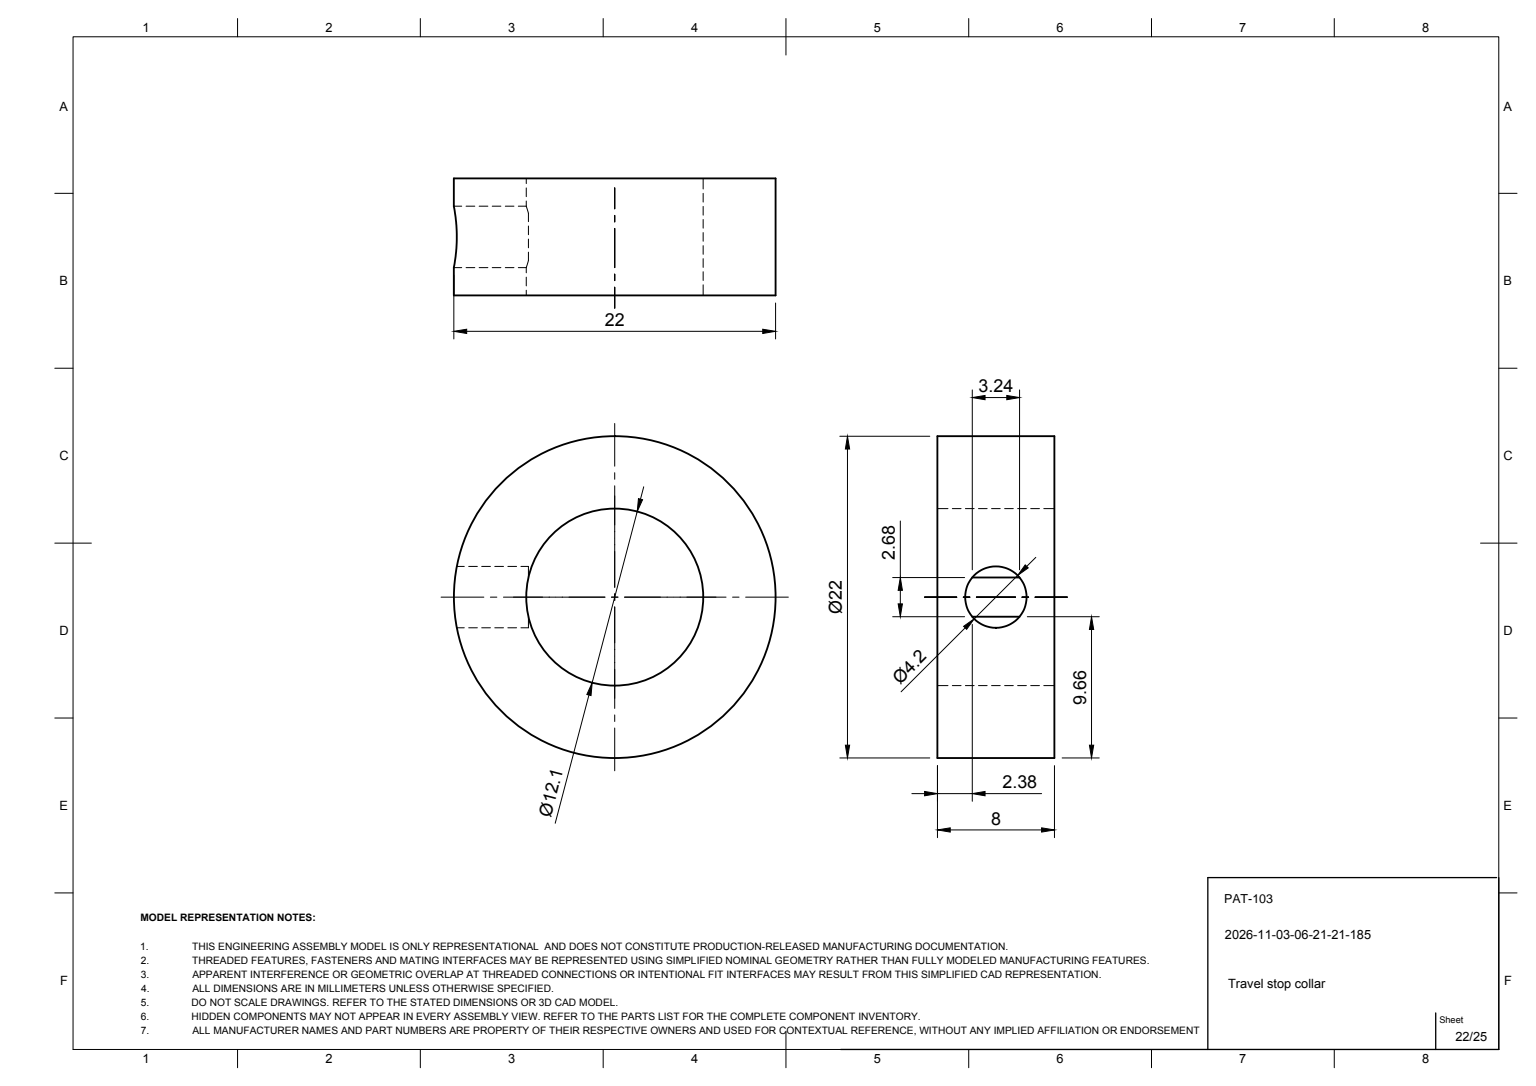
ISO-10303-21;
HEADER;
/* Generated by software containing ST-Developer
 * from STEP Tools, Inc. (www.steptools.com) 
 */

FILE_DESCRIPTION(
/* description */ ('Telescoping shaft support with lock collar'),
/* implementation_level */ '2;1');

FILE_NAME(
/* name */ 'Travel stop collar.step',
/* time_stamp */ '2026-10-27T10:48:51-07:00',
/* author */ (''),
/* organization */ (''),
/* preprocessor_version */ 'ST-DEVELOPER v20.2',
/* originating_system */ 'Autodesk Translation Framework v15.17.0.0',
/* authorisation */ '');

FILE_SCHEMA (('AUTOMOTIVE_DESIGN { 1 0 10303 214 3 1 1 }'));
ENDSEC;

DATA;
#10=MECHANICAL_DESIGN_GEOMETRIC_PRESENTATION_REPRESENTATION('',(#255),#7349);
#187=B_SPLINE_CURVE_WITH_KNOTS('',3,(#6910,#6911,#6912,#6913,#6914,#6915),
 .UNSPECIFIED.,.F.,.F.,(4,2,4),(0.818088904349175,0.878131747417171,0.957937926194042),
 .UNSPECIFIED.);
#188=B_SPLINE_CURVE_WITH_KNOTS('',3,(#6919,#6920,#6921,#6922,#6923,#6924),
 .UNSPECIFIED.,.F.,.F.,(4,2,4),(0.319312642064681,0.399118820841551,0.459161663909547),
 .UNSPECIFIED.);
#189=B_SPLINE_CURVE_WITH_KNOTS('',3,(#6925,#6926,#6927,#6928,#6929,#6930),
 .UNSPECIFIED.,.F.,.F.,(4,2,4),(0.179463620219814,0.23950646328781,0.319312642064681),
 .UNSPECIFIED.);
#190=B_SPLINE_CURVE_WITH_KNOTS('',3,(#6931,#6932,#6933,#6934,#6935,#6936),
 .UNSPECIFIED.,.F.,.F.,(4,2,4),(0.957937926194042,1.03774410497091,1.09778694803891),
 .UNSPECIFIED.);
#191=B_SPLINE_CURVE_WITH_KNOTS('',3,(#6940,#6941,#6942,#6943,#6944,#6945,
#6946,#6947,#6948,#6949),.UNSPECIFIED.,.F.,.F.,(4,2,2,2,4),(0.,0.0793157643915228,
0.158631528783046,0.237943615933651,0.317255703084257),.UNSPECIFIED.);
#192=B_SPLINE_CURVE_WITH_KNOTS('',3,(#6951,#6952,#6953,#6954,#6955,#6956,
#6957,#6958,#6959,#6960),.UNSPECIFIED.,.F.,.F.,(4,2,2,2,4),(0.951767109252772,
1.03107919640338,1.11039128355398,1.18970704794551,1.26902281233703),
 .UNSPECIFIED.);
#193=B_SPLINE_CURVE_WITH_KNOTS('',3,(#6961,#6962,#6963,#6964,#6965,#6966,
#6967,#6968,#6969,#6970,#6971,#6972,#6973,#6974,#6975,#6976,#6977,#6978),
 .UNSPECIFIED.,.F.,.F.,(4,2,2,2,2,2,2,2,4),(0.317255703084257,0.396567790234863,
0.475879877385469,0.555195641776992,0.634511406168514,0.713827170560037,
0.79314293495156,0.872455022102166,0.951767109252772),.UNSPECIFIED.);
#215=SHAPE_REPRESENTATION_RELATIONSHIP('SRR','None',#7459,#235);
#235=ADVANCED_BREP_SHAPE_REPRESENTATION('',(#274),#7343);
#255=STYLED_ITEM('',(#7641),#274);
#274=MANIFOLD_SOLID_BREP('Body1',#3979);
#349=FACE_BOUND('',#967,.T.);
#350=FACE_BOUND('',#969,.T.);
#461=PLANE('',#4573);
#462=PLANE('',#4577);
#463=PLANE('',#4584);
#464=PLANE('',#4585);
#665=FACE_OUTER_BOUND('',#961,.T.);
#666=FACE_OUTER_BOUND('',#962,.T.);
#667=FACE_OUTER_BOUND('',#963,.T.);
#668=FACE_OUTER_BOUND('',#964,.T.);
#669=FACE_OUTER_BOUND('',#965,.T.);
#670=FACE_OUTER_BOUND('',#966,.T.);
#671=FACE_OUTER_BOUND('',#968,.T.);
#961=EDGE_LOOP('',(#3428,#3429));
#962=EDGE_LOOP('',(#3430,#3431,#3432,#3433,#3434,#3435,#3436,#3437,#3438,
#3439,#3440));
#963=EDGE_LOOP('',(#3441,#3442));
#964=EDGE_LOOP('',(#3443,#3444,#3445,#3446,#3447,#3448,#3449,#3450,#3451,
#3452,#3453,#3454));
#965=EDGE_LOOP('',(#3455,#3456,#3457,#3458,#3459,#3460,#3461,#3462,#3463));
#966=EDGE_LOOP('',(#3464));
#967=EDGE_LOOP('',(#3465));
#968=EDGE_LOOP('',(#3466));
#969=EDGE_LOOP('',(#3467));
#1241=LINE('',#6905,#1521);
#1242=LINE('',#6938,#1522);
#1243=LINE('',#6980,#1523);
#1244=LINE('',#6984,#1524);
#1245=LINE('',#6986,#1525);
#1246=LINE('',#6991,#1526);
#1247=LINE('',#6993,#1527);
#1521=VECTOR('',#5655,1.);
#1522=VECTOR('',#5662,0.210000000000001);
#1523=VECTOR('',#5665,1.);
#1524=VECTOR('',#5670,0.605);
#1525=VECTOR('',#5671,0.605);
#1526=VECTOR('',#5678,1.1);
#1527=VECTOR('',#5679,1.1);
#1762=CIRCLE('',#4574,0.210000000000001);
#1763=CIRCLE('',#4576,0.210000000000001);
#1764=CIRCLE('',#4579,0.605);
#1765=CIRCLE('',#4580,0.605);
#1766=CIRCLE('',#4582,1.1);
#1767=CIRCLE('',#4583,1.1);
#2059=VERTEX_POINT('',#6903);
#2060=VERTEX_POINT('',#6904);
#2061=VERTEX_POINT('',#6908);
#2062=VERTEX_POINT('',#6909);
#2063=VERTEX_POINT('',#6916);
#2064=VERTEX_POINT('',#6918);
#2065=VERTEX_POINT('',#6937);
#2066=VERTEX_POINT('',#6939);
#2067=VERTEX_POINT('',#6950);
#2068=VERTEX_POINT('',#6982);
#2069=VERTEX_POINT('',#6985);
#2070=VERTEX_POINT('',#6989);
#2071=VERTEX_POINT('',#6992);
#2526=EDGE_CURVE('',#2059,#2060,#1241,.T.);
#2527=EDGE_CURVE('',#2059,#2060,#1762,.T.);
#2528=EDGE_CURVE('',#2061,#2062,#187,.T.);
#2529=EDGE_CURVE('',#2063,#2061,#1763,.T.);
#2530=EDGE_CURVE('',#2064,#2063,#188,.T.);
#2531=EDGE_CURVE('',#2060,#2064,#189,.T.);
#2532=EDGE_CURVE('',#2062,#2059,#190,.T.);
#2533=EDGE_CURVE('',#2062,#2065,#1242,.T.);
#2534=EDGE_CURVE('',#2066,#2065,#191,.T.);
#2535=EDGE_CURVE('',#2067,#2066,#192,.T.);
#2536=EDGE_CURVE('',#2065,#2067,#193,.T.);
#2537=EDGE_CURVE('',#2063,#2061,#1243,.T.);
#2538=EDGE_CURVE('',#2068,#2068,#1764,.T.);
#2539=EDGE_CURVE('',#2068,#2064,#1244,.T.);
#2540=EDGE_CURVE('',#2062,#2069,#1245,.T.);
#2541=EDGE_CURVE('',#2069,#2069,#1765,.T.);
#2542=EDGE_CURVE('',#2070,#2070,#1766,.T.);
#2543=EDGE_CURVE('',#2070,#2067,#1246,.T.);
#2544=EDGE_CURVE('',#2065,#2071,#1247,.T.);
#2545=EDGE_CURVE('',#2071,#2071,#1767,.T.);
#3428=ORIENTED_EDGE('',*,*,#2526,.F.);
#3429=ORIENTED_EDGE('',*,*,#2527,.T.);
#3430=ORIENTED_EDGE('',*,*,#2528,.F.);
#3431=ORIENTED_EDGE('',*,*,#2529,.F.);
#3432=ORIENTED_EDGE('',*,*,#2530,.F.);
#3433=ORIENTED_EDGE('',*,*,#2531,.F.);
#3434=ORIENTED_EDGE('',*,*,#2527,.F.);
#3435=ORIENTED_EDGE('',*,*,#2532,.F.);
#3436=ORIENTED_EDGE('',*,*,#2533,.T.);
#3437=ORIENTED_EDGE('',*,*,#2534,.F.);
#3438=ORIENTED_EDGE('',*,*,#2535,.F.);
#3439=ORIENTED_EDGE('',*,*,#2536,.F.);
#3440=ORIENTED_EDGE('',*,*,#2533,.F.);
#3441=ORIENTED_EDGE('',*,*,#2537,.F.);
#3442=ORIENTED_EDGE('',*,*,#2529,.T.);
#3443=ORIENTED_EDGE('',*,*,#2538,.F.);
#3444=ORIENTED_EDGE('',*,*,#2539,.T.);
#3445=ORIENTED_EDGE('',*,*,#2530,.T.);
#3446=ORIENTED_EDGE('',*,*,#2537,.T.);
#3447=ORIENTED_EDGE('',*,*,#2528,.T.);
#3448=ORIENTED_EDGE('',*,*,#2540,.T.);
#3449=ORIENTED_EDGE('',*,*,#2541,.T.);
#3450=ORIENTED_EDGE('',*,*,#2540,.F.);
#3451=ORIENTED_EDGE('',*,*,#2532,.T.);
#3452=ORIENTED_EDGE('',*,*,#2526,.T.);
#3453=ORIENTED_EDGE('',*,*,#2531,.T.);
#3454=ORIENTED_EDGE('',*,*,#2539,.F.);
#3455=ORIENTED_EDGE('',*,*,#2542,.F.);
#3456=ORIENTED_EDGE('',*,*,#2543,.T.);
#3457=ORIENTED_EDGE('',*,*,#2535,.T.);
#3458=ORIENTED_EDGE('',*,*,#2534,.T.);
#3459=ORIENTED_EDGE('',*,*,#2544,.T.);
#3460=ORIENTED_EDGE('',*,*,#2545,.T.);
#3461=ORIENTED_EDGE('',*,*,#2544,.F.);
#3462=ORIENTED_EDGE('',*,*,#2536,.T.);
#3463=ORIENTED_EDGE('',*,*,#2543,.F.);
#3464=ORIENTED_EDGE('',*,*,#2542,.T.);
#3465=ORIENTED_EDGE('',*,*,#2538,.T.);
#3466=ORIENTED_EDGE('',*,*,#2545,.F.);
#3467=ORIENTED_EDGE('',*,*,#2541,.F.);
#3724=CYLINDRICAL_SURFACE('',#4575,0.210000000000001);
#3725=CYLINDRICAL_SURFACE('',#4578,0.605);
#3726=CYLINDRICAL_SURFACE('',#4581,1.1);
#3908=ADVANCED_FACE('',(#665),#461,.T.);
#3909=ADVANCED_FACE('',(#666),#3724,.F.);
#3910=ADVANCED_FACE('',(#667),#462,.T.);
#3911=ADVANCED_FACE('',(#668),#3725,.F.);
#3912=ADVANCED_FACE('',(#669),#3726,.T.);
#3913=ADVANCED_FACE('',(#670,#349),#463,.T.);
#3914=ADVANCED_FACE('',(#671,#350),#464,.F.);
#3979=CLOSED_SHELL('',(#3908,#3909,#3910,#3911,#3912,#3913,#3914));
#4572=AXIS2_PLACEMENT_3D('',#6901,#5651,#5652);
#4573=AXIS2_PLACEMENT_3D('',#6902,#5653,#5654);
#4574=AXIS2_PLACEMENT_3D('',#6906,#5656,#5657);
#4575=AXIS2_PLACEMENT_3D('',#6907,#5658,#5659);
#4576=AXIS2_PLACEMENT_3D('',#6917,#5660,#5661);
#4577=AXIS2_PLACEMENT_3D('',#6979,#5663,#5664);
#4578=AXIS2_PLACEMENT_3D('',#6981,#5666,#5667);
#4579=AXIS2_PLACEMENT_3D('',#6983,#5668,#5669);
#4580=AXIS2_PLACEMENT_3D('',#6987,#5672,#5673);
#4581=AXIS2_PLACEMENT_3D('',#6988,#5674,#5675);
#4582=AXIS2_PLACEMENT_3D('',#6990,#5676,#5677);
#4583=AXIS2_PLACEMENT_3D('',#6994,#5680,#5681);
#4584=AXIS2_PLACEMENT_3D('',#6995,#5682,#5683);
#4585=AXIS2_PLACEMENT_3D('',#6996,#5684,#5685);
#5651=DIRECTION('axis',(0.,0.,1.));
#5652=DIRECTION('refdir',(1.,0.,0.));
#5653=DIRECTION('center_axis',(0.,0.,1.));
#5654=DIRECTION('ref_axis',(1.,0.,0.));
#5655=DIRECTION('',(1.,0.,0.));
#5656=DIRECTION('center_axis',(0.,0.,1.));
#5657=DIRECTION('ref_axis',(1.,0.,0.));
#5658=DIRECTION('center_axis',(0.,0.,1.));
#5659=DIRECTION('ref_axis',(1.,0.,0.));
#5660=DIRECTION('center_axis',(0.,0.,1.));
#5661=DIRECTION('ref_axis',(1.,0.,0.));
#5662=DIRECTION('',(0.,0.,1.));
#5663=DIRECTION('center_axis',(0.,0.,1.));
#5664=DIRECTION('ref_axis',(1.,0.,0.));
#5665=DIRECTION('',(-1.,0.,0.));
#5666=DIRECTION('center_axis',(1.,0.,0.));
#5667=DIRECTION('ref_axis',(0.,0.,-1.));
#5668=DIRECTION('center_axis',(-1.,0.,0.));
#5669=DIRECTION('ref_axis',(0.,0.,-1.));
#5670=DIRECTION('',(-1.,0.,0.));
#5671=DIRECTION('',(-1.,0.,0.));
#5672=DIRECTION('center_axis',(-1.,0.,0.));
#5673=DIRECTION('ref_axis',(0.,0.,-1.));
#5674=DIRECTION('center_axis',(1.,0.,0.));
#5675=DIRECTION('ref_axis',(0.,0.,-1.));
#5676=DIRECTION('center_axis',(1.,0.,0.));
#5677=DIRECTION('ref_axis',(0.,0.,-1.));
#5678=DIRECTION('',(-1.,0.,0.));
#5679=DIRECTION('',(-1.,0.,0.));
#5680=DIRECTION('center_axis',(1.,0.,0.));
#5681=DIRECTION('ref_axis',(0.,0.,-1.));
#5682=DIRECTION('center_axis',(1.,0.,0.));
#5683=DIRECTION('ref_axis',(0.,0.,-1.));
#5684=DIRECTION('center_axis',(1.,0.,0.));
#5685=DIRECTION('ref_axis',(0.,0.,-1.));
#6901=CARTESIAN_POINT('',(0.,0.,0.));
#6902=CARTESIAN_POINT('Origin',(-17.3,0.,4.09));
#6903=CARTESIAN_POINT('',(-17.4617868968736,-0.133884278389959,4.09));
#6904=CARTESIAN_POINT('',(-17.1382131031264,-0.133884278389959,4.09));
#6905=CARTESIAN_POINT('',(-17.7,-0.133884278389959,4.09));
#6906=CARTESIAN_POINT('Origin',(-17.3,0.,4.09));
#6907=CARTESIAN_POINT('Origin',(-17.3,0.,4.09));
#6908=CARTESIAN_POINT('',(-17.4617868968736,0.133884278389959,4.09));
#6909=CARTESIAN_POINT('',(-17.51,7.73468293597467E-17,4.105));
#6910=CARTESIAN_POINT('Ctrl Pts',(-17.4617868968736,0.133884278389958,4.09));
#6911=CARTESIAN_POINT('Ctrl Pts',(-17.4747211682176,0.118254395260802,4.09354677224418));
#6912=CARTESIAN_POINT('Ctrl Pts',(-17.4857993165874,0.100109787682302,4.09698224789957));
#6913=CARTESIAN_POINT('Ctrl Pts',(-17.5046385610544,0.0548298721325208,
4.1030741628997));
#6914=CARTESIAN_POINT('Ctrl Pts',(-17.51,0.0266020595922901,4.105));
#6915=CARTESIAN_POINT('Ctrl Pts',(-17.51,-1.73472347597681E-16,4.105));
#6916=CARTESIAN_POINT('',(-17.1382131031264,0.133884278389959,4.09));
#6917=CARTESIAN_POINT('Origin',(-17.3,0.,4.09));
#6918=CARTESIAN_POINT('',(-17.09,-2.66372248183466E-17,4.105));
#6919=CARTESIAN_POINT('Ctrl Pts',(-17.09,1.04083408558608E-16,4.105));
#6920=CARTESIAN_POINT('Ctrl Pts',(-17.09,0.0266020595922904,4.105));
#6921=CARTESIAN_POINT('Ctrl Pts',(-17.0953614389456,0.0548298721325207,
4.1030741628997));
#6922=CARTESIAN_POINT('Ctrl Pts',(-17.1142006834126,0.100109787682302,4.09698224789957));
#6923=CARTESIAN_POINT('Ctrl Pts',(-17.1252788317824,0.118254395260807,4.09354677224418));
#6924=CARTESIAN_POINT('Ctrl Pts',(-17.1382131031264,0.133884278389958,4.09));
#6925=CARTESIAN_POINT('Ctrl Pts',(-17.1382131031264,-0.13388427838996,4.09));
#6926=CARTESIAN_POINT('Ctrl Pts',(-17.1252788317824,-0.118254395260808,
4.09354677224418));
#6927=CARTESIAN_POINT('Ctrl Pts',(-17.1142006834126,-0.100109787682302,
4.09698224789957));
#6928=CARTESIAN_POINT('Ctrl Pts',(-17.0953614389456,-0.0548298721325207,
4.1030741628997));
#6929=CARTESIAN_POINT('Ctrl Pts',(-17.09,-0.0266020595922903,4.105));
#6930=CARTESIAN_POINT('Ctrl Pts',(-17.09,-4.16333634234434E-17,4.105));
#6931=CARTESIAN_POINT('Ctrl Pts',(-17.51,1.87350135405495E-16,4.105));
#6932=CARTESIAN_POINT('Ctrl Pts',(-17.51,-0.0266020595922901,4.105));
#6933=CARTESIAN_POINT('Ctrl Pts',(-17.5046385610544,-0.0548298721325207,
4.1030741628997));
#6934=CARTESIAN_POINT('Ctrl Pts',(-17.4857993165874,-0.100109787682302,
4.09698224789957));
#6935=CARTESIAN_POINT('Ctrl Pts',(-17.4747211682176,-0.118254395260802,
4.09354677224418));
#6936=CARTESIAN_POINT('Ctrl Pts',(-17.4617868968736,-0.133884278389957,
4.09));
#6937=CARTESIAN_POINT('',(-17.51,-2.57175827820945E-17,4.6));
#6938=CARTESIAN_POINT('',(-17.51,-2.57175827820945E-17,4.09));
#6939=CARTESIAN_POINT('',(-17.3,-0.210000000000001,4.57976849370594));
#6940=CARTESIAN_POINT('Ctrl Pts',(-17.3,-0.210000000000001,4.57976849370594));
#6941=CARTESIAN_POINT('Ctrl Pts',(-17.3264385881305,-0.21,4.57976849370594));
#6942=CARTESIAN_POINT('Ctrl Pts',(-17.3545937812549,-0.204702922670978,
4.58084015664674));
#6943=CARTESIAN_POINT('Ctrl Pts',(-17.4063134455413,-0.183251796806355,
4.58468313707126));
#6944=CARTESIAN_POINT('Ctrl Pts',(-17.4298836707411,-0.167101177357215,
4.58739593054622));
#6945=CARTESIAN_POINT('Ctrl Pts',(-17.4671003146174,-0.129884533480966,
4.59246633289124));
#6946=CARTESIAN_POINT('Ctrl Pts',(-17.4832516101634,-0.106313940757288,
4.59515738895358));
#6947=CARTESIAN_POINT('Ctrl Pts',(-17.5047032265697,-0.0545930033295209,
4.59895039220591));
#6948=CARTESIAN_POINT('Ctrl Pts',(-17.51,-0.0264373623835352,4.6));
#6949=CARTESIAN_POINT('Ctrl Pts',(-17.51,6.24500451351651E-17,4.6));
#6950=CARTESIAN_POINT('',(-17.09,-5.00083391933364E-17,4.6));
#6951=CARTESIAN_POINT('Ctrl Pts',(-17.09,3.46944695195361E-17,4.6));
#6952=CARTESIAN_POINT('Ctrl Pts',(-17.09,-0.0264373623835353,4.6));
#6953=CARTESIAN_POINT('Ctrl Pts',(-17.0952967734303,-0.0545930033295208,
4.59895039220591));
#6954=CARTESIAN_POINT('Ctrl Pts',(-17.1167483898366,-0.106313940757288,
4.59515738895358));
#6955=CARTESIAN_POINT('Ctrl Pts',(-17.1328996853826,-0.129884533480966,
4.59246633289124));
#6956=CARTESIAN_POINT('Ctrl Pts',(-17.1701163292589,-0.167101177357215,
4.58739593054622));
#6957=CARTESIAN_POINT('Ctrl Pts',(-17.1936865544587,-0.183251796806355,
4.58468313707126));
#6958=CARTESIAN_POINT('Ctrl Pts',(-17.2454062187451,-0.204702922670978,
4.58084015664674));
#6959=CARTESIAN_POINT('Ctrl Pts',(-17.2735614118695,-0.210000000000001,
4.57976849370594));
#6960=CARTESIAN_POINT('Ctrl Pts',(-17.3,-0.210000000000001,4.57976849370594));
#6961=CARTESIAN_POINT('Ctrl Pts',(-17.51,-9.71445146547012E-17,4.6));
#6962=CARTESIAN_POINT('Ctrl Pts',(-17.51,0.0264373623835352,4.6));
#6963=CARTESIAN_POINT('Ctrl Pts',(-17.5047032265697,0.0545930033295208,
4.59895039220591));
#6964=CARTESIAN_POINT('Ctrl Pts',(-17.4832516101634,0.106313940757288,4.59515738895358));
#6965=CARTESIAN_POINT('Ctrl Pts',(-17.4671003146174,0.129884533480966,4.59246633289124));
#6966=CARTESIAN_POINT('Ctrl Pts',(-17.4298836707411,0.167101177357215,4.58739593054622));
#6967=CARTESIAN_POINT('Ctrl Pts',(-17.4063134455413,0.183251796806355,4.58468313707126));
#6968=CARTESIAN_POINT('Ctrl Pts',(-17.3545937812549,0.204702922670978,4.58084015664674));
#6969=CARTESIAN_POINT('Ctrl Pts',(-17.3264385881305,0.210000000000001,4.57976849370594));
#6970=CARTESIAN_POINT('Ctrl Pts',(-17.2735614118695,0.210000000000001,4.57976849370594));
#6971=CARTESIAN_POINT('Ctrl Pts',(-17.2454062187451,0.204702922670978,4.58084015664674));
#6972=CARTESIAN_POINT('Ctrl Pts',(-17.1936865544587,0.183251796806355,4.58468313707126));
#6973=CARTESIAN_POINT('Ctrl Pts',(-17.1701163292589,0.167101177357215,4.58739593054622));
#6974=CARTESIAN_POINT('Ctrl Pts',(-17.1328996853826,0.129884533480966,4.59246633289124));
#6975=CARTESIAN_POINT('Ctrl Pts',(-17.1167483898366,0.106313940757288,4.59515738895358));
#6976=CARTESIAN_POINT('Ctrl Pts',(-17.0952967734303,0.0545930033295209,
4.59895039220591));
#6977=CARTESIAN_POINT('Ctrl Pts',(-17.09,0.0264373623835352,4.6));
#6978=CARTESIAN_POINT('Ctrl Pts',(-17.09,-1.11022302462516E-16,4.6));
#6979=CARTESIAN_POINT('Origin',(-17.3,0.,4.09));
#6980=CARTESIAN_POINT('',(-17.7,0.133884278389959,4.09));
#6981=CARTESIAN_POINT('Origin',(-17.7,0.,3.5));
#6982=CARTESIAN_POINT('',(-16.9,-7.40911313484149E-17,4.105));
#6983=CARTESIAN_POINT('Origin',(-16.9,0.,3.5));
#6984=CARTESIAN_POINT('',(-17.7,-7.40911313484149E-17,4.105));
#6985=CARTESIAN_POINT('',(-17.7,-7.40911313484149E-17,4.105));
#6986=CARTESIAN_POINT('',(-17.7,-7.40911313484149E-17,4.105));
#6987=CARTESIAN_POINT('Origin',(-17.7,0.,3.5));
#6988=CARTESIAN_POINT('Origin',(-17.7,0.,3.5));
#6989=CARTESIAN_POINT('',(-16.9,-1.34711147906209E-16,4.6));
#6990=CARTESIAN_POINT('Origin',(-16.9,0.,3.5));
#6991=CARTESIAN_POINT('',(-17.7,-1.34711147906209E-16,4.6));
#6992=CARTESIAN_POINT('',(-17.7,-1.34711147906209E-16,4.6));
#6993=CARTESIAN_POINT('',(-17.7,-1.34711147906209E-16,4.6));
#6994=CARTESIAN_POINT('Origin',(-17.7,0.,3.5));
#6995=CARTESIAN_POINT('Origin',(-16.9,0.,3.5));
#6996=CARTESIAN_POINT('Origin',(-17.7,0.,3.5));
#7318=UNCERTAINTY_MEASURE_WITH_UNIT(LENGTH_MEASURE(0.001),#7350,
'DISTANCE_ACCURACY_VALUE',
'Maximum model space distance between geometric entities at asserted c
onnectivities');
#7324=UNCERTAINTY_MEASURE_WITH_UNIT(LENGTH_MEASURE(0.001),#7350,
'DISTANCE_ACCURACY_VALUE',
'Maximum model space distance between geometric entities at asserted c
onnectivities');
#7343=(
GEOMETRIC_REPRESENTATION_CONTEXT(3)
GLOBAL_UNCERTAINTY_ASSIGNED_CONTEXT((#7318))
GLOBAL_UNIT_ASSIGNED_CONTEXT((#7350,#7352,#7353))
REPRESENTATION_CONTEXT('','3D')
);
#7349=(
GEOMETRIC_REPRESENTATION_CONTEXT(3)
GLOBAL_UNCERTAINTY_ASSIGNED_CONTEXT((#7324))
GLOBAL_UNIT_ASSIGNED_CONTEXT((#7350,#7352,#7353))
REPRESENTATION_CONTEXT('','3D')
);
#7350=(
LENGTH_UNIT()
NAMED_UNIT(*)
SI_UNIT(.CENTI.,.METRE.)
);
#7352=(
NAMED_UNIT(*)
PLANE_ANGLE_UNIT()
SI_UNIT($,.RADIAN.)
);
#7353=(
NAMED_UNIT(*)
SI_UNIT($,.STERADIAN.)
SOLID_ANGLE_UNIT()
);
#7372=SHAPE_DEFINITION_REPRESENTATION(#7398,#7459);
#7398=PRODUCT_DEFINITION_SHAPE('',$,#7484);
#7459=SHAPE_REPRESENTATION('',(#4572),#7343);
#7465=PRODUCT_DEFINITION_CONTEXT('part definition',#7539,'design');
#7484=PRODUCT_DEFINITION('Travel stop collar','Travel stop collar',#7508,
#7465);
#7508=PRODUCT_DEFINITION_FORMATION('',$,#7559);
#7539=APPLICATION_CONTEXT(
'Core Data for Automotive Mechanical Design Process');
#7540=PRODUCT_CONTEXT('part definition',#7539,'mechanical');
#7559=PRODUCT('Travel stop collar','Travel stop collar',
'Travel stop collar',(#7540));
#7635=COLOUR_RGB('Off White',0.89,0.88,0.83);
#7636=FILL_AREA_STYLE_COLOUR('',#7635);
#7637=FILL_AREA_STYLE('',(#7636));
#7638=SURFACE_STYLE_FILL_AREA(#7637);
#7639=SURFACE_SIDE_STYLE('',(#7638));
#7640=SURFACE_STYLE_USAGE(.BOTH.,#7639);
#7641=PRESENTATION_STYLE_ASSIGNMENT((#7640));
ENDSEC;
END-ISO-10303-21;
